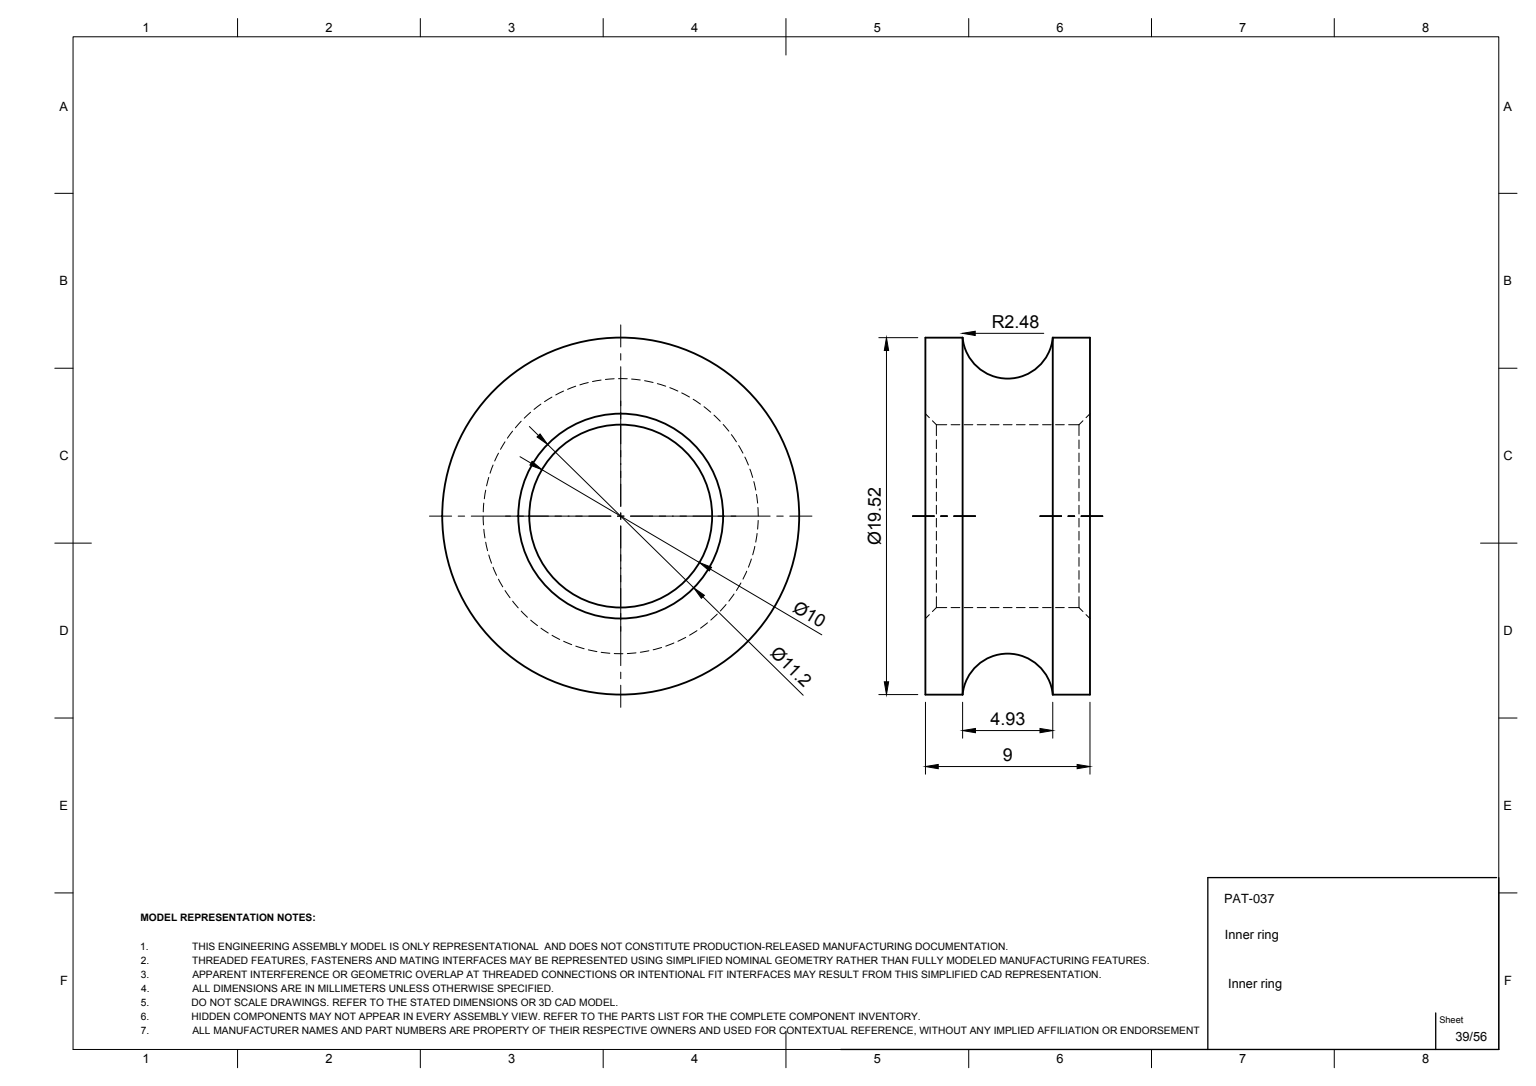
ISO-10303-21;
HEADER;
/* Generated by software containing ST-Developer
 * from STEP Tools, Inc. (www.steptools.com) 
 */

FILE_DESCRIPTION(
/* description */ ('Flywheel Crank-Slider'),
/* implementation_level */ '2;1');

FILE_NAME(
/* name */ 'Inner ring.step',
/* time_stamp */ '2026-10-28T03:23:13-07:00',
/* author */ (''),
/* organization */ (''),
/* preprocessor_version */ 'ST-DEVELOPER v20.2',
/* originating_system */ 'Autodesk Translation Framework v15.17.0.0',
/* authorisation */ '');

FILE_SCHEMA (('AUTOMOTIVE_DESIGN { 1 0 10303 214 3 1 1 }'));
ENDSEC;

DATA;
#10=MECHANICAL_DESIGN_GEOMETRIC_PRESENTATION_REPRESENTATION('',(#706),#17322);
#11=TOROIDAL_SURFACE('',#10395,1.,0.247676);
#552=CONICAL_SURFACE('',#10406,0.53,0.785398163397448);
#553=CONICAL_SURFACE('',#10413,0.53,0.785398163397448);
#601=SHAPE_REPRESENTATION_RELATIONSHIP('SRR','None',#17601,#653);
#653=ADVANCED_BREP_SHAPE_REPRESENTATION('',(#763),#17305);
#706=STYLED_ITEM('',(#17931),#763);
#763=MANIFOLD_SOLID_BREP('Body1',#9088);
#943=FACE_BOUND('',#2400,.T.);
#944=FACE_BOUND('',#2403,.T.);
#1242=PLANE('',#10408);
#1243=PLANE('',#10411);
#1702=FACE_OUTER_BOUND('',#2395,.T.);
#1703=FACE_OUTER_BOUND('',#2396,.T.);
#1704=FACE_OUTER_BOUND('',#2397,.T.);
#1705=FACE_OUTER_BOUND('',#2398,.T.);
#1706=FACE_OUTER_BOUND('',#2399,.T.);
#1707=FACE_OUTER_BOUND('',#2401,.T.);
#1708=FACE_OUTER_BOUND('',#2402,.T.);
#1709=FACE_OUTER_BOUND('',#2404,.T.);
#2395=EDGE_LOOP('',(#7698,#7699,#7700,#7701,#7702,#7703));
#2396=EDGE_LOOP('',(#7704,#7705,#7706,#7707,#7708));
#2397=EDGE_LOOP('',(#7709,#7710,#7711,#7712));
#2398=EDGE_LOOP('',(#7713,#7714,#7715,#7716));
#2399=EDGE_LOOP('',(#7717));
#2400=EDGE_LOOP('',(#7718));
#2401=EDGE_LOOP('',(#7719,#7720,#7721,#7722,#7723));
#2402=EDGE_LOOP('',(#7724));
#2403=EDGE_LOOP('',(#7725));
#2404=EDGE_LOOP('',(#7726,#7727,#7728,#7729));
#3086=LINE('',#16062,#3697);
#3087=LINE('',#16068,#3698);
#3088=LINE('',#16072,#3699);
#3089=LINE('',#16078,#3700);
#3090=LINE('',#16083,#3701);
#3697=VECTOR('',#12734,0.976185);
#3698=VECTOR('',#12741,0.5);
#3699=VECTOR('',#12746,0.53);
#3700=VECTOR('',#12755,0.976185);
#3701=VECTOR('',#12762,0.53);
#4120=CIRCLE('',#10396,0.976185);
#4121=CIRCLE('',#10397,0.976185);
#4122=CIRCLE('',#10398,0.247676);
#4123=CIRCLE('',#10399,0.976185);
#4124=CIRCLE('',#10400,0.976185);
#4125=CIRCLE('',#10402,0.976185);
#4126=CIRCLE('',#10404,0.5);
#4127=CIRCLE('',#10405,0.5);
#4128=CIRCLE('',#10407,0.56);
#4129=CIRCLE('',#10410,0.976185);
#4130=CIRCLE('',#10412,0.56);
#4799=VERTEX_POINT('',#16051);
#4800=VERTEX_POINT('',#16052);
#4801=VERTEX_POINT('',#16055);
#4802=VERTEX_POINT('',#16057);
#4803=VERTEX_POINT('',#16061);
#4804=VERTEX_POINT('',#16065);
#4805=VERTEX_POINT('',#16067);
#4806=VERTEX_POINT('',#16071);
#4807=VERTEX_POINT('',#16076);
#4808=VERTEX_POINT('',#16080);
#5806=EDGE_CURVE('',#4799,#4800,#4120,.T.);
#5807=EDGE_CURVE('',#4800,#4799,#4121,.T.);
#5808=EDGE_CURVE('',#4800,#4801,#4122,.T.);
#5809=EDGE_CURVE('',#4802,#4801,#4123,.T.);
#5810=EDGE_CURVE('',#4801,#4802,#4124,.T.);
#5811=EDGE_CURVE('',#4802,#4803,#3086,.T.);
#5812=EDGE_CURVE('',#4803,#4803,#4125,.T.);
#5813=EDGE_CURVE('',#4804,#4804,#4126,.T.);
#5814=EDGE_CURVE('',#4804,#4805,#3087,.T.);
#5815=EDGE_CURVE('',#4805,#4805,#4127,.T.);
#5816=EDGE_CURVE('',#4805,#4806,#3088,.T.);
#5817=EDGE_CURVE('',#4806,#4806,#4128,.T.);
#5818=EDGE_CURVE('',#4807,#4807,#4129,.T.);
#5819=EDGE_CURVE('',#4807,#4799,#3089,.T.);
#5820=EDGE_CURVE('',#4808,#4808,#4130,.T.);
#5821=EDGE_CURVE('',#4808,#4804,#3090,.T.);
#7698=ORIENTED_EDGE('',*,*,#5806,.F.);
#7699=ORIENTED_EDGE('',*,*,#5807,.F.);
#7700=ORIENTED_EDGE('',*,*,#5808,.T.);
#7701=ORIENTED_EDGE('',*,*,#5809,.F.);
#7702=ORIENTED_EDGE('',*,*,#5810,.F.);
#7703=ORIENTED_EDGE('',*,*,#5808,.F.);
#7704=ORIENTED_EDGE('',*,*,#5809,.T.);
#7705=ORIENTED_EDGE('',*,*,#5810,.T.);
#7706=ORIENTED_EDGE('',*,*,#5811,.T.);
#7707=ORIENTED_EDGE('',*,*,#5812,.T.);
#7708=ORIENTED_EDGE('',*,*,#5811,.F.);
#7709=ORIENTED_EDGE('',*,*,#5813,.T.);
#7710=ORIENTED_EDGE('',*,*,#5814,.T.);
#7711=ORIENTED_EDGE('',*,*,#5815,.F.);
#7712=ORIENTED_EDGE('',*,*,#5814,.F.);
#7713=ORIENTED_EDGE('',*,*,#5815,.T.);
#7714=ORIENTED_EDGE('',*,*,#5816,.T.);
#7715=ORIENTED_EDGE('',*,*,#5817,.F.);
#7716=ORIENTED_EDGE('',*,*,#5816,.F.);
#7717=ORIENTED_EDGE('',*,*,#5812,.F.);
#7718=ORIENTED_EDGE('',*,*,#5817,.T.);
#7719=ORIENTED_EDGE('',*,*,#5818,.F.);
#7720=ORIENTED_EDGE('',*,*,#5819,.T.);
#7721=ORIENTED_EDGE('',*,*,#5806,.T.);
#7722=ORIENTED_EDGE('',*,*,#5807,.T.);
#7723=ORIENTED_EDGE('',*,*,#5819,.F.);
#7724=ORIENTED_EDGE('',*,*,#5818,.T.);
#7725=ORIENTED_EDGE('',*,*,#5820,.F.);
#7726=ORIENTED_EDGE('',*,*,#5820,.T.);
#7727=ORIENTED_EDGE('',*,*,#5821,.T.);
#7728=ORIENTED_EDGE('',*,*,#5813,.F.);
#7729=ORIENTED_EDGE('',*,*,#5821,.F.);
#8461=CYLINDRICAL_SURFACE('',#10401,0.976185);
#8462=CYLINDRICAL_SURFACE('',#10403,0.5);
#8463=CYLINDRICAL_SURFACE('',#10409,0.976185);
#8893=ADVANCED_FACE('',(#1702),#11,.F.);
#8894=ADVANCED_FACE('',(#1703),#8461,.T.);
#8895=ADVANCED_FACE('',(#1704),#8462,.F.);
#8896=ADVANCED_FACE('',(#1705),#552,.F.);
#8897=ADVANCED_FACE('',(#1706,#943),#1242,.T.);
#8898=ADVANCED_FACE('',(#1707),#8463,.T.);
#8899=ADVANCED_FACE('',(#1708,#944),#1243,.T.);
#8900=ADVANCED_FACE('',(#1709),#553,.F.);
#9088=CLOSED_SHELL('',(#8893,#8894,#8895,#8896,#8897,#8898,#8899,#8900));
#10394=AXIS2_PLACEMENT_3D('',#16049,#12718,#12719);
#10395=AXIS2_PLACEMENT_3D('',#16050,#12720,#12721);
#10396=AXIS2_PLACEMENT_3D('',#16053,#12722,#12723);
#10397=AXIS2_PLACEMENT_3D('',#16054,#12724,#12725);
#10398=AXIS2_PLACEMENT_3D('',#16056,#12726,#12727);
#10399=AXIS2_PLACEMENT_3D('',#16058,#12728,#12729);
#10400=AXIS2_PLACEMENT_3D('',#16059,#12730,#12731);
#10401=AXIS2_PLACEMENT_3D('',#16060,#12732,#12733);
#10402=AXIS2_PLACEMENT_3D('',#16063,#12735,#12736);
#10403=AXIS2_PLACEMENT_3D('',#16064,#12737,#12738);
#10404=AXIS2_PLACEMENT_3D('',#16066,#12739,#12740);
#10405=AXIS2_PLACEMENT_3D('',#16069,#12742,#12743);
#10406=AXIS2_PLACEMENT_3D('',#16070,#12744,#12745);
#10407=AXIS2_PLACEMENT_3D('',#16073,#12747,#12748);
#10408=AXIS2_PLACEMENT_3D('',#16074,#12749,#12750);
#10409=AXIS2_PLACEMENT_3D('',#16075,#12751,#12752);
#10410=AXIS2_PLACEMENT_3D('',#16077,#12753,#12754);
#10411=AXIS2_PLACEMENT_3D('',#16079,#12756,#12757);
#10412=AXIS2_PLACEMENT_3D('',#16081,#12758,#12759);
#10413=AXIS2_PLACEMENT_3D('',#16082,#12760,#12761);
#12718=DIRECTION('axis',(0.,0.,1.));
#12719=DIRECTION('refdir',(1.,0.,0.));
#12720=DIRECTION('center_axis',(0.,-1.,0.));
#12721=DIRECTION('ref_axis',(0.,0.,-1.));
#12722=DIRECTION('center_axis',(0.,-1.,0.));
#12723=DIRECTION('ref_axis',(1.,0.,0.));
#12724=DIRECTION('center_axis',(0.,-1.,0.));
#12725=DIRECTION('ref_axis',(1.,0.,0.));
#12726=DIRECTION('center_axis',(1.,0.,1.22464679914735E-16));
#12727=DIRECTION('ref_axis',(-1.22464679914735E-16,0.,1.));
#12728=DIRECTION('center_axis',(0.,1.,0.));
#12729=DIRECTION('ref_axis',(1.,0.,0.));
#12730=DIRECTION('center_axis',(0.,1.,0.));
#12731=DIRECTION('ref_axis',(1.,0.,0.));
#12732=DIRECTION('center_axis',(0.,-1.,0.));
#12733=DIRECTION('ref_axis',(1.,0.,0.));
#12734=DIRECTION('',(0.,1.,0.));
#12735=DIRECTION('center_axis',(0.,-1.,0.));
#12736=DIRECTION('ref_axis',(1.,0.,0.));
#12737=DIRECTION('center_axis',(0.,-1.,0.));
#12738=DIRECTION('ref_axis',(1.,0.,0.));
#12739=DIRECTION('center_axis',(0.,-1.,0.));
#12740=DIRECTION('ref_axis',(1.,0.,0.));
#12741=DIRECTION('',(0.,1.,0.));
#12742=DIRECTION('center_axis',(0.,-1.,0.));
#12743=DIRECTION('ref_axis',(1.,0.,0.));
#12744=DIRECTION('center_axis',(0.,1.,0.));
#12745=DIRECTION('ref_axis',(1.,0.,0.));
#12746=DIRECTION('',(-0.707106781186547,0.707106781186548,-8.65956056235493E-17));
#12747=DIRECTION('center_axis',(0.,-1.,0.));
#12748=DIRECTION('ref_axis',(1.,0.,0.));
#12749=DIRECTION('center_axis',(0.,1.,0.));
#12750=DIRECTION('ref_axis',(0.,0.,1.));
#12751=DIRECTION('center_axis',(0.,-1.,0.));
#12752=DIRECTION('ref_axis',(1.,0.,0.));
#12753=DIRECTION('center_axis',(0.,-1.,0.));
#12754=DIRECTION('ref_axis',(1.,0.,0.));
#12755=DIRECTION('',(0.,1.,0.));
#12756=DIRECTION('center_axis',(0.,-1.,0.));
#12757=DIRECTION('ref_axis',(0.,0.,-1.));
#12758=DIRECTION('center_axis',(0.,-1.,0.));
#12759=DIRECTION('ref_axis',(1.,0.,0.));
#12760=DIRECTION('center_axis',(0.,-1.,0.));
#12761=DIRECTION('ref_axis',(1.,0.,0.));
#12762=DIRECTION('',(0.707106781186547,0.707106781186548,8.65956056235493E-17));
#16049=CARTESIAN_POINT('',(0.,0.,0.));
#16050=CARTESIAN_POINT('Origin',(0.,0.,0.));
#16051=CARTESIAN_POINT('',(-0.976185,-0.246528389340863,-1.19548183562566E-16));
#16052=CARTESIAN_POINT('',(-1.19548183562566E-16,-0.246528389340863,0.976185));
#16053=CARTESIAN_POINT('Origin',(0.,-0.246528389340863,0.));
#16054=CARTESIAN_POINT('Origin',(0.,-0.246528389340863,0.));
#16055=CARTESIAN_POINT('',(-1.19548183562566E-16,0.246528389340863,0.976185));
#16056=CARTESIAN_POINT('Origin',(-1.22464679914735E-16,0.,1.));
#16057=CARTESIAN_POINT('',(-0.976185,0.246528389340863,1.19548183562566E-16));
#16058=CARTESIAN_POINT('Origin',(0.,0.246528389340863,0.));
#16059=CARTESIAN_POINT('Origin',(0.,0.246528389340863,0.));
#16060=CARTESIAN_POINT('Origin',(0.,0.,0.));
#16061=CARTESIAN_POINT('',(-0.976185,0.45,-1.19548183562566E-16));
#16062=CARTESIAN_POINT('',(-0.976185,0.,-1.19548183562566E-16));
#16063=CARTESIAN_POINT('Origin',(0.,0.45,0.));
#16064=CARTESIAN_POINT('Origin',(0.,0.,0.));
#16065=CARTESIAN_POINT('',(-0.5,-0.39,-6.12323399573677E-17));
#16066=CARTESIAN_POINT('Origin',(0.,-0.39,0.));
#16067=CARTESIAN_POINT('',(-0.5,0.39,-6.12323399573677E-17));
#16068=CARTESIAN_POINT('',(-0.5,0.,-6.12323399573677E-17));
#16069=CARTESIAN_POINT('Origin',(0.,0.39,0.));
#16070=CARTESIAN_POINT('Origin',(0.,0.42,0.));
#16071=CARTESIAN_POINT('',(-0.56,0.45,-6.85802207522518E-17));
#16072=CARTESIAN_POINT('',(-0.53,0.42,-6.49062803548097E-17));
#16073=CARTESIAN_POINT('Origin',(0.,0.45,0.));
#16074=CARTESIAN_POINT('Origin',(0.976185,0.45,0.));
#16075=CARTESIAN_POINT('Origin',(0.,0.,0.));
#16076=CARTESIAN_POINT('',(-0.976185,-0.45,-1.19548183562566E-16));
#16077=CARTESIAN_POINT('Origin',(0.,-0.45,0.));
#16078=CARTESIAN_POINT('',(-0.976185,0.,-1.19548183562566E-16));
#16079=CARTESIAN_POINT('Origin',(0.56,-0.45,0.));
#16080=CARTESIAN_POINT('',(-0.56,-0.45,-6.85802207522518E-17));
#16081=CARTESIAN_POINT('Origin',(0.,-0.45,0.));
#16082=CARTESIAN_POINT('Origin',(0.,-0.42,0.));
#16083=CARTESIAN_POINT('',(-0.53,-0.42,-6.49062803548097E-17));
#17244=UNCERTAINTY_MEASURE_WITH_UNIT(LENGTH_MEASURE(0.001),#17323,
'DISTANCE_ACCURACY_VALUE',
'Maximum model space distance between geometric entities at asserted c
onnectivities');
#17261=UNCERTAINTY_MEASURE_WITH_UNIT(LENGTH_MEASURE(0.001),#17323,
'DISTANCE_ACCURACY_VALUE',
'Maximum model space distance between geometric entities at asserted c
onnectivities');
#17305=(
GEOMETRIC_REPRESENTATION_CONTEXT(3)
GLOBAL_UNCERTAINTY_ASSIGNED_CONTEXT((#17244))
GLOBAL_UNIT_ASSIGNED_CONTEXT((#17323,#17325,#17326))
REPRESENTATION_CONTEXT('','3D')
);
#17322=(
GEOMETRIC_REPRESENTATION_CONTEXT(3)
GLOBAL_UNCERTAINTY_ASSIGNED_CONTEXT((#17261))
GLOBAL_UNIT_ASSIGNED_CONTEXT((#17323,#17325,#17326))
REPRESENTATION_CONTEXT('','3D')
);
#17323=(
LENGTH_UNIT()
NAMED_UNIT(*)
SI_UNIT(.CENTI.,.METRE.)
);
#17325=(
NAMED_UNIT(*)
PLANE_ANGLE_UNIT()
SI_UNIT($,.RADIAN.)
);
#17326=(
NAMED_UNIT(*)
SI_UNIT($,.STERADIAN.)
SOLID_ANGLE_UNIT()
);
#17370=SHAPE_DEFINITION_REPRESENTATION(#17432,#17601);
#17432=PRODUCT_DEFINITION_SHAPE('',$,#17662);
#17601=SHAPE_REPRESENTATION('',(#10394),#17305);
#17618=PRODUCT_DEFINITION_CONTEXT('part definition',#17800,'design');
#17662=PRODUCT_DEFINITION('Inner ring','Inner ring',#17722,#17618);
#17722=PRODUCT_DEFINITION_FORMATION('',$,#17845);
#17800=APPLICATION_CONTEXT(
'Core Data for Automotive Mechanical Design Process');
#17801=PRODUCT_CONTEXT('part definition',#17800,'mechanical');
#17845=PRODUCT('Inner ring','Inner ring','Inner ring',(#17801));
#17925=COLOUR_RGB('Grey',0.48,0.52,0.57);
#17926=FILL_AREA_STYLE_COLOUR('',#17925);
#17927=FILL_AREA_STYLE('',(#17926));
#17928=SURFACE_STYLE_FILL_AREA(#17927);
#17929=SURFACE_SIDE_STYLE('',(#17928));
#17930=SURFACE_STYLE_USAGE(.BOTH.,#17929);
#17931=PRESENTATION_STYLE_ASSIGNMENT((#17930));
ENDSEC;
END-ISO-10303-21;
